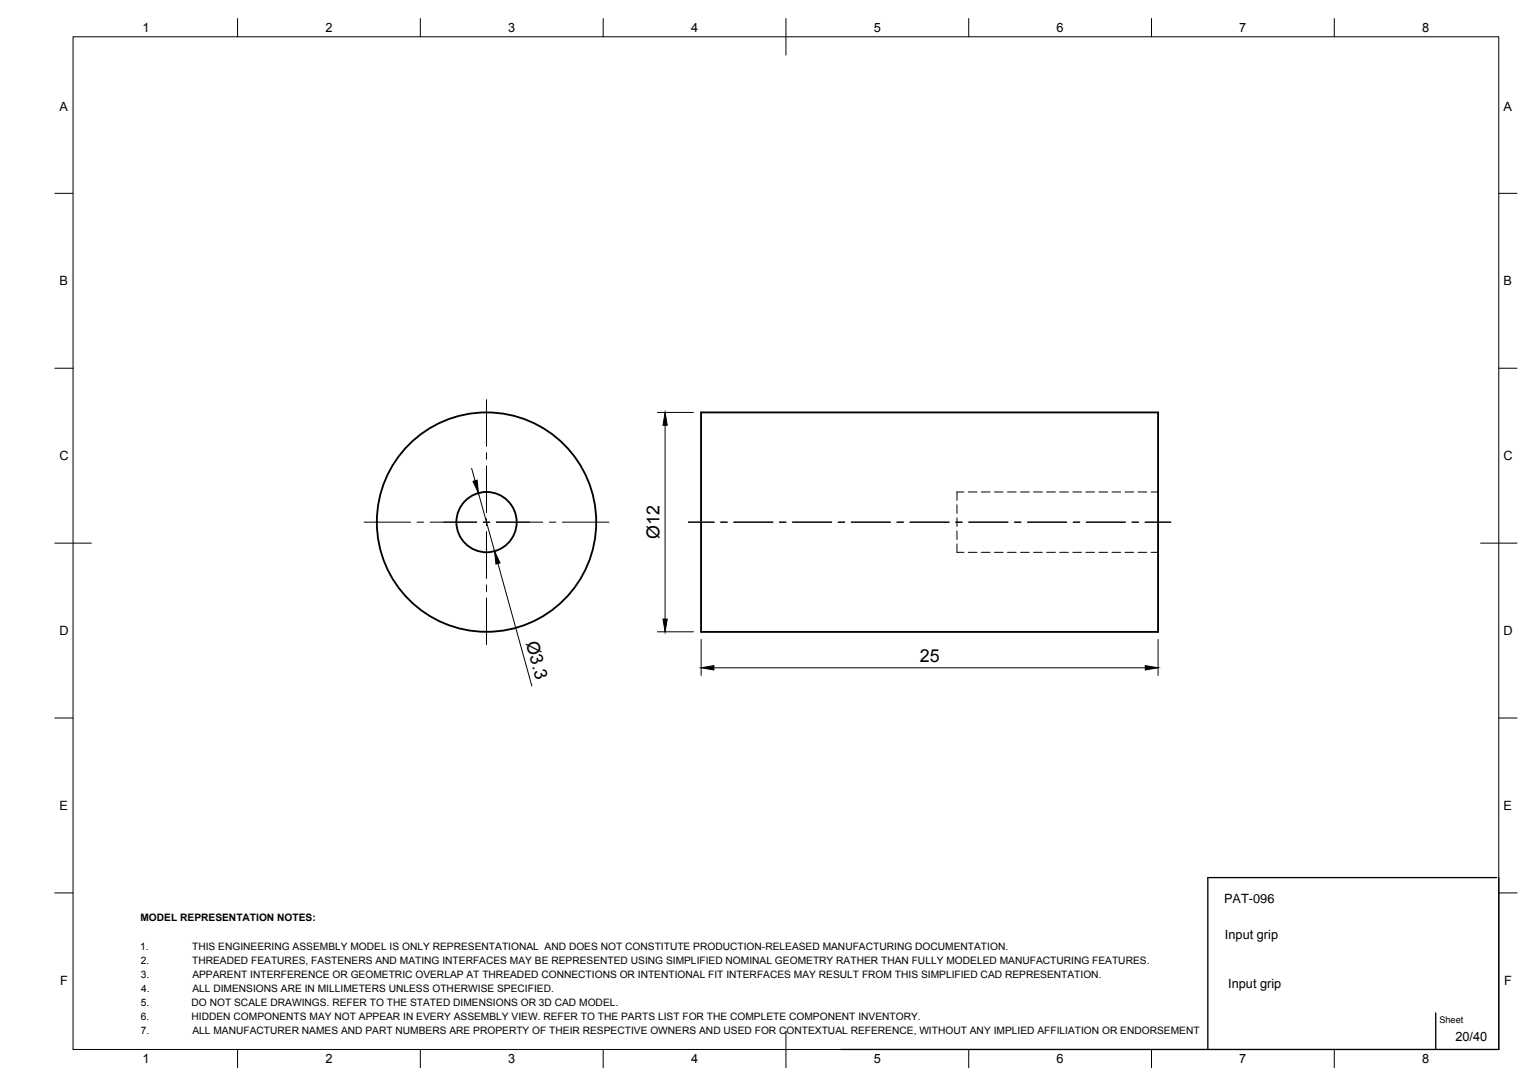
ISO-10303-21;
HEADER;
/* Generated by software containing ST-Developer
 * from STEP Tools, Inc. (www.steptools.com) 
 */

FILE_DESCRIPTION(
/* description */ ('PAT-096'),
/* implementation_level */ '2;1');

FILE_NAME(
/* name */ 'Input grip.step',
/* time_stamp */ '2026-10-29T17:03:14-07:00',
/* author */ (''),
/* organization */ (''),
/* preprocessor_version */ 'ST-DEVELOPER v20.2',
/* originating_system */ 'Autodesk Translation Framework v15.17.0.0',
/* authorisation */ '');

FILE_SCHEMA (('AUTOMOTIVE_DESIGN { 1 0 10303 214 3 1 1 }'));
ENDSEC;

DATA;
#10=MECHANICAL_DESIGN_GEOMETRIC_PRESENTATION_REPRESENTATION('',(#419),#10650);
#349=SHAPE_REPRESENTATION_RELATIONSHIP('SRR','None',#10811,#380);
#380=ADVANCED_BREP_SHAPE_REPRESENTATION('',(#457),#10629);
#419=STYLED_ITEM('',(#11071),#457);
#457=MANIFOLD_SOLID_BREP('Body1',#5553);
#550=FACE_BOUND('',#1389,.T.);
#696=PLANE('',#6321);
#697=PLANE('',#6325);
#698=PLANE('',#6326);
#971=FACE_OUTER_BOUND('',#1384,.T.);
#972=FACE_OUTER_BOUND('',#1385,.T.);
#973=FACE_OUTER_BOUND('',#1386,.T.);
#974=FACE_OUTER_BOUND('',#1387,.T.);
#975=FACE_OUTER_BOUND('',#1388,.T.);
#1384=EDGE_LOOP('',(#4493,#4494,#4495,#4496));
#1385=EDGE_LOOP('',(#4497));
#1386=EDGE_LOOP('',(#4498,#4499,#4500,#4501));
#1387=EDGE_LOOP('',(#4502));
#1388=EDGE_LOOP('',(#4503));
#1389=EDGE_LOOP('',(#4504));
#1765=LINE('',#9802,#2094);
#1766=LINE('',#9809,#2095);
#2094=VECTOR('',#7645,0.165);
#2095=VECTOR('',#7654,0.6);
#2458=CIRCLE('',#6319,0.165);
#2459=CIRCLE('',#6320,0.165);
#2460=CIRCLE('',#6323,0.6);
#2461=CIRCLE('',#6324,0.6);
#2845=VERTEX_POINT('',#9799);
#2846=VERTEX_POINT('',#9801);
#2847=VERTEX_POINT('',#9806);
#2848=VERTEX_POINT('',#9808);
#3425=EDGE_CURVE('',#2845,#2845,#2458,.T.);
#3426=EDGE_CURVE('',#2845,#2846,#1765,.T.);
#3427=EDGE_CURVE('',#2846,#2846,#2459,.T.);
#3428=EDGE_CURVE('',#2847,#2847,#2460,.T.);
#3429=EDGE_CURVE('',#2847,#2848,#1766,.T.);
#3430=EDGE_CURVE('',#2848,#2848,#2461,.T.);
#4493=ORIENTED_EDGE('',*,*,#3425,.F.);
#4494=ORIENTED_EDGE('',*,*,#3426,.T.);
#4495=ORIENTED_EDGE('',*,*,#3427,.T.);
#4496=ORIENTED_EDGE('',*,*,#3426,.F.);
#4497=ORIENTED_EDGE('',*,*,#3427,.F.);
#4498=ORIENTED_EDGE('',*,*,#3428,.F.);
#4499=ORIENTED_EDGE('',*,*,#3429,.T.);
#4500=ORIENTED_EDGE('',*,*,#3430,.T.);
#4501=ORIENTED_EDGE('',*,*,#3429,.F.);
#4502=ORIENTED_EDGE('',*,*,#3428,.T.);
#4503=ORIENTED_EDGE('',*,*,#3430,.F.);
#4504=ORIENTED_EDGE('',*,*,#3425,.T.);
#5142=CYLINDRICAL_SURFACE('',#6318,0.165);
#5143=CYLINDRICAL_SURFACE('',#6322,0.6);
#5376=ADVANCED_FACE('',(#971),#5142,.F.);
#5377=ADVANCED_FACE('',(#972),#696,.F.);
#5378=ADVANCED_FACE('',(#973),#5143,.T.);
#5379=ADVANCED_FACE('',(#974),#697,.T.);
#5380=ADVANCED_FACE('',(#975,#550),#698,.F.);
#5553=CLOSED_SHELL('',(#5376,#5377,#5378,#5379,#5380));
#6317=AXIS2_PLACEMENT_3D('',#9797,#7639,#7640);
#6318=AXIS2_PLACEMENT_3D('',#9798,#7641,#7642);
#6319=AXIS2_PLACEMENT_3D('',#9800,#7643,#7644);
#6320=AXIS2_PLACEMENT_3D('',#9803,#7646,#7647);
#6321=AXIS2_PLACEMENT_3D('',#9804,#7648,#7649);
#6322=AXIS2_PLACEMENT_3D('',#9805,#7650,#7651);
#6323=AXIS2_PLACEMENT_3D('',#9807,#7652,#7653);
#6324=AXIS2_PLACEMENT_3D('',#9810,#7655,#7656);
#6325=AXIS2_PLACEMENT_3D('',#9811,#7657,#7658);
#6326=AXIS2_PLACEMENT_3D('',#9812,#7659,#7660);
#7639=DIRECTION('axis',(0.,0.,1.));
#7640=DIRECTION('refdir',(1.,0.,0.));
#7641=DIRECTION('center_axis',(0.,0.,1.));
#7642=DIRECTION('ref_axis',(1.,0.,0.));
#7643=DIRECTION('center_axis',(0.,0.,1.));
#7644=DIRECTION('ref_axis',(1.,0.,0.));
#7645=DIRECTION('',(0.,0.,1.));
#7646=DIRECTION('center_axis',(0.,0.,1.));
#7647=DIRECTION('ref_axis',(1.,0.,0.));
#7648=DIRECTION('center_axis',(0.,0.,1.));
#7649=DIRECTION('ref_axis',(1.,0.,0.));
#7650=DIRECTION('center_axis',(0.,0.,1.));
#7651=DIRECTION('ref_axis',(1.,0.,0.));
#7652=DIRECTION('center_axis',(0.,0.,1.));
#7653=DIRECTION('ref_axis',(1.,0.,0.));
#7654=DIRECTION('',(0.,0.,-1.));
#7655=DIRECTION('center_axis',(0.,0.,1.));
#7656=DIRECTION('ref_axis',(1.,0.,0.));
#7657=DIRECTION('center_axis',(0.,0.,1.));
#7658=DIRECTION('ref_axis',(1.,0.,0.));
#7659=DIRECTION('center_axis',(0.,0.,1.));
#7660=DIRECTION('ref_axis',(1.,0.,0.));
#9797=CARTESIAN_POINT('',(0.,0.,0.));
#9798=CARTESIAN_POINT('Origin',(-2.5,-2.5,5.5));
#9799=CARTESIAN_POINT('',(-2.665,-2.5,5.6));
#9800=CARTESIAN_POINT('Origin',(-2.5,-2.5,5.6));
#9801=CARTESIAN_POINT('',(-2.665,-2.5,6.7));
#9802=CARTESIAN_POINT('',(-2.665,-2.5,5.5));
#9803=CARTESIAN_POINT('Origin',(-2.5,-2.5,6.7));
#9804=CARTESIAN_POINT('Origin',(-2.5,-2.5,6.7));
#9805=CARTESIAN_POINT('Origin',(-2.5,-2.5,5.6));
#9806=CARTESIAN_POINT('',(-3.1,-2.5,8.1));
#9807=CARTESIAN_POINT('Origin',(-2.5,-2.5,8.1));
#9808=CARTESIAN_POINT('',(-3.1,-2.5,5.6));
#9809=CARTESIAN_POINT('',(-3.1,-2.5,5.6));
#9810=CARTESIAN_POINT('Origin',(-2.5,-2.5,5.6));
#9811=CARTESIAN_POINT('Origin',(-2.5,-2.5,8.1));
#9812=CARTESIAN_POINT('Origin',(-2.5,-2.5,5.6));
#10590=UNCERTAINTY_MEASURE_WITH_UNIT(LENGTH_MEASURE(0.001),#10651,
'DISTANCE_ACCURACY_VALUE',
'Maximum model space distance between geometric entities at asserted c
onnectivities');
#10611=UNCERTAINTY_MEASURE_WITH_UNIT(LENGTH_MEASURE(0.001),#10651,
'DISTANCE_ACCURACY_VALUE',
'Maximum model space distance between geometric entities at asserted c
onnectivities');
#10629=(
GEOMETRIC_REPRESENTATION_CONTEXT(3)
GLOBAL_UNCERTAINTY_ASSIGNED_CONTEXT((#10590))
GLOBAL_UNIT_ASSIGNED_CONTEXT((#10651,#10653,#10654))
REPRESENTATION_CONTEXT('','3D')
);
#10650=(
GEOMETRIC_REPRESENTATION_CONTEXT(3)
GLOBAL_UNCERTAINTY_ASSIGNED_CONTEXT((#10611))
GLOBAL_UNIT_ASSIGNED_CONTEXT((#10651,#10653,#10654))
REPRESENTATION_CONTEXT('','3D')
);
#10651=(
LENGTH_UNIT()
NAMED_UNIT(*)
SI_UNIT(.CENTI.,.METRE.)
);
#10653=(
NAMED_UNIT(*)
PLANE_ANGLE_UNIT()
SI_UNIT($,.RADIAN.)
);
#10654=(
NAMED_UNIT(*)
SI_UNIT($,.STERADIAN.)
SOLID_ANGLE_UNIT()
);
#10672=SHAPE_DEFINITION_REPRESENTATION(#10715,#10811);
#10715=PRODUCT_DEFINITION_SHAPE('',$,#10850);
#10811=SHAPE_REPRESENTATION('',(#6317),#10629);
#10832=PRODUCT_DEFINITION_CONTEXT('part definition',#10948,'design');
#10850=PRODUCT_DEFINITION('Input grip','Input grip',#10888,#10832);
#10888=PRODUCT_DEFINITION_FORMATION('',$,#10967);
#10948=APPLICATION_CONTEXT(
'Core Data for Automotive Mechanical Design Process');
#10949=PRODUCT_CONTEXT('part definition',#10948,'mechanical');
#10967=PRODUCT('Input grip','Input grip','Input grip',(#10949));
#11065=COLOUR_RGB('Black',0.12,0.14,0.17);
#11066=FILL_AREA_STYLE_COLOUR('',#11065);
#11067=FILL_AREA_STYLE('',(#11066));
#11068=SURFACE_STYLE_FILL_AREA(#11067);
#11069=SURFACE_SIDE_STYLE('',(#11068));
#11070=SURFACE_STYLE_USAGE(.BOTH.,#11069);
#11071=PRESENTATION_STYLE_ASSIGNMENT((#11070));
ENDSEC;
END-ISO-10303-21;
